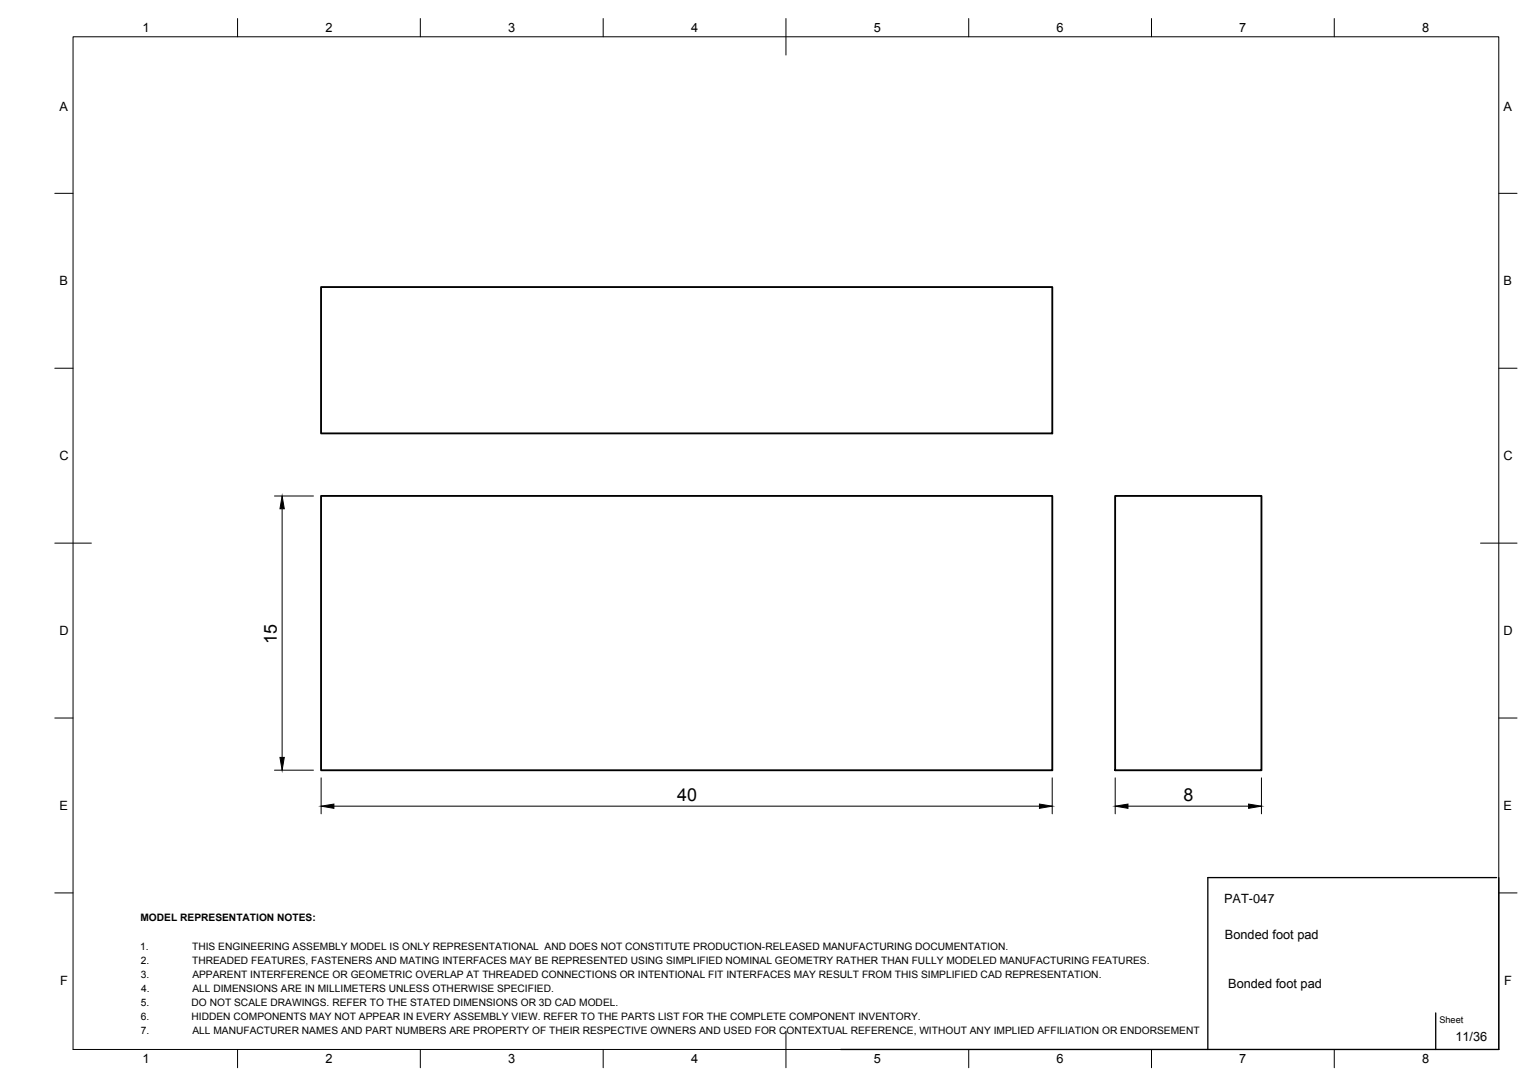
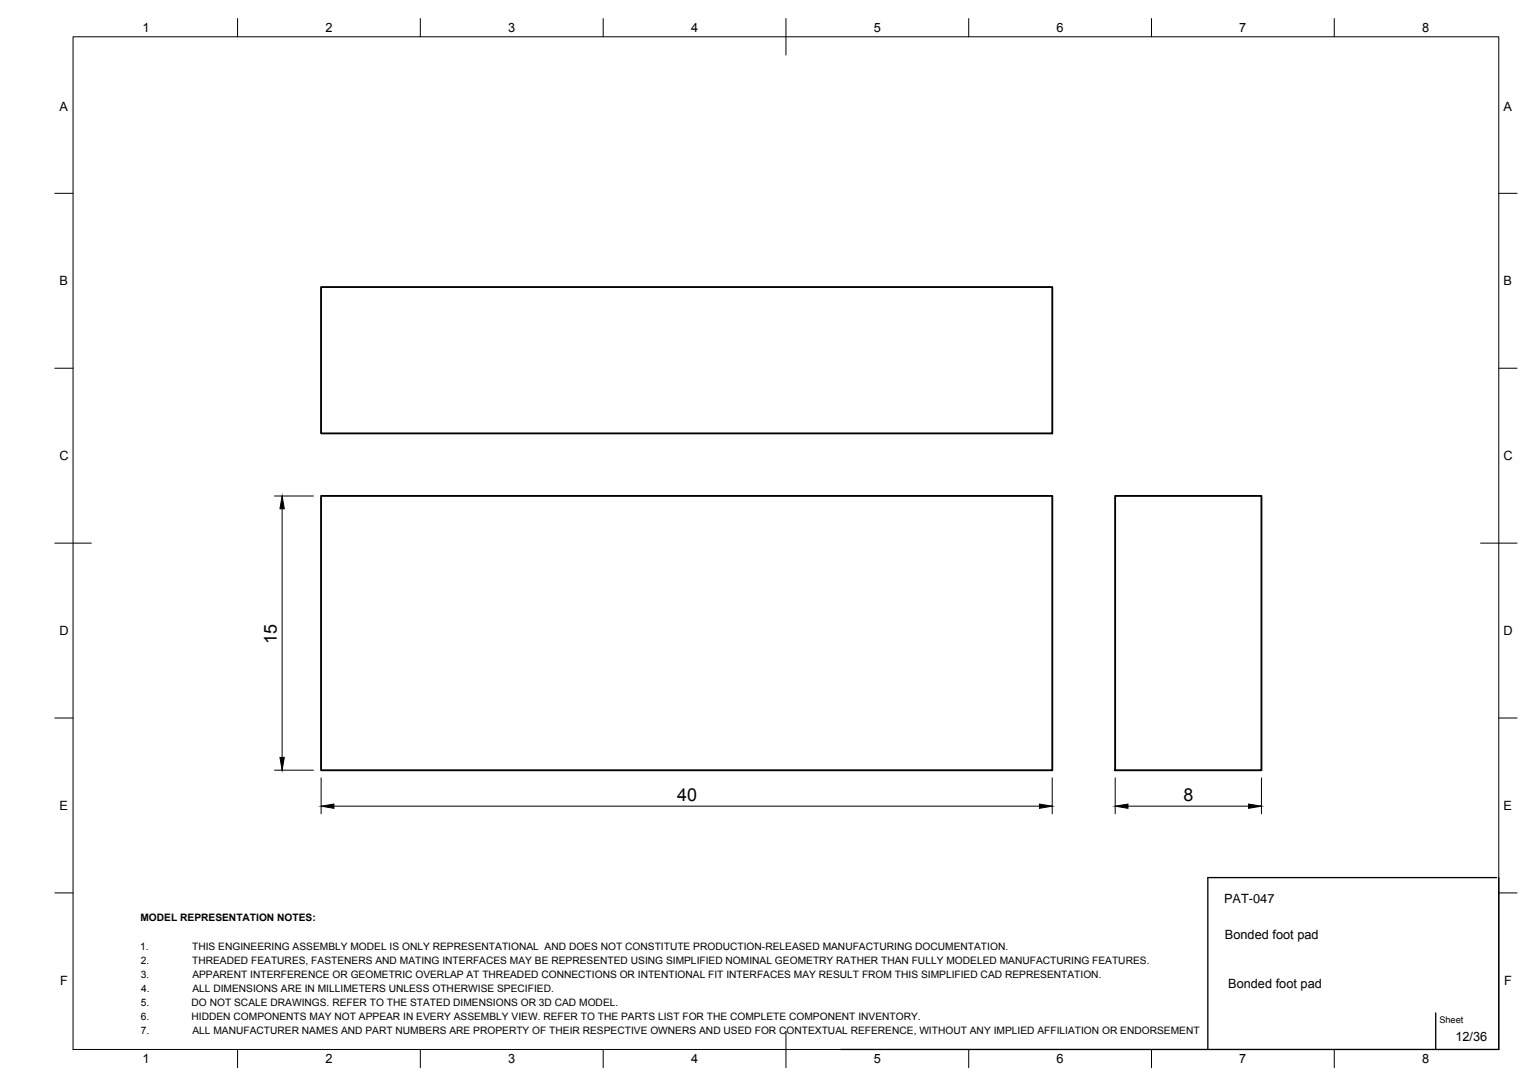
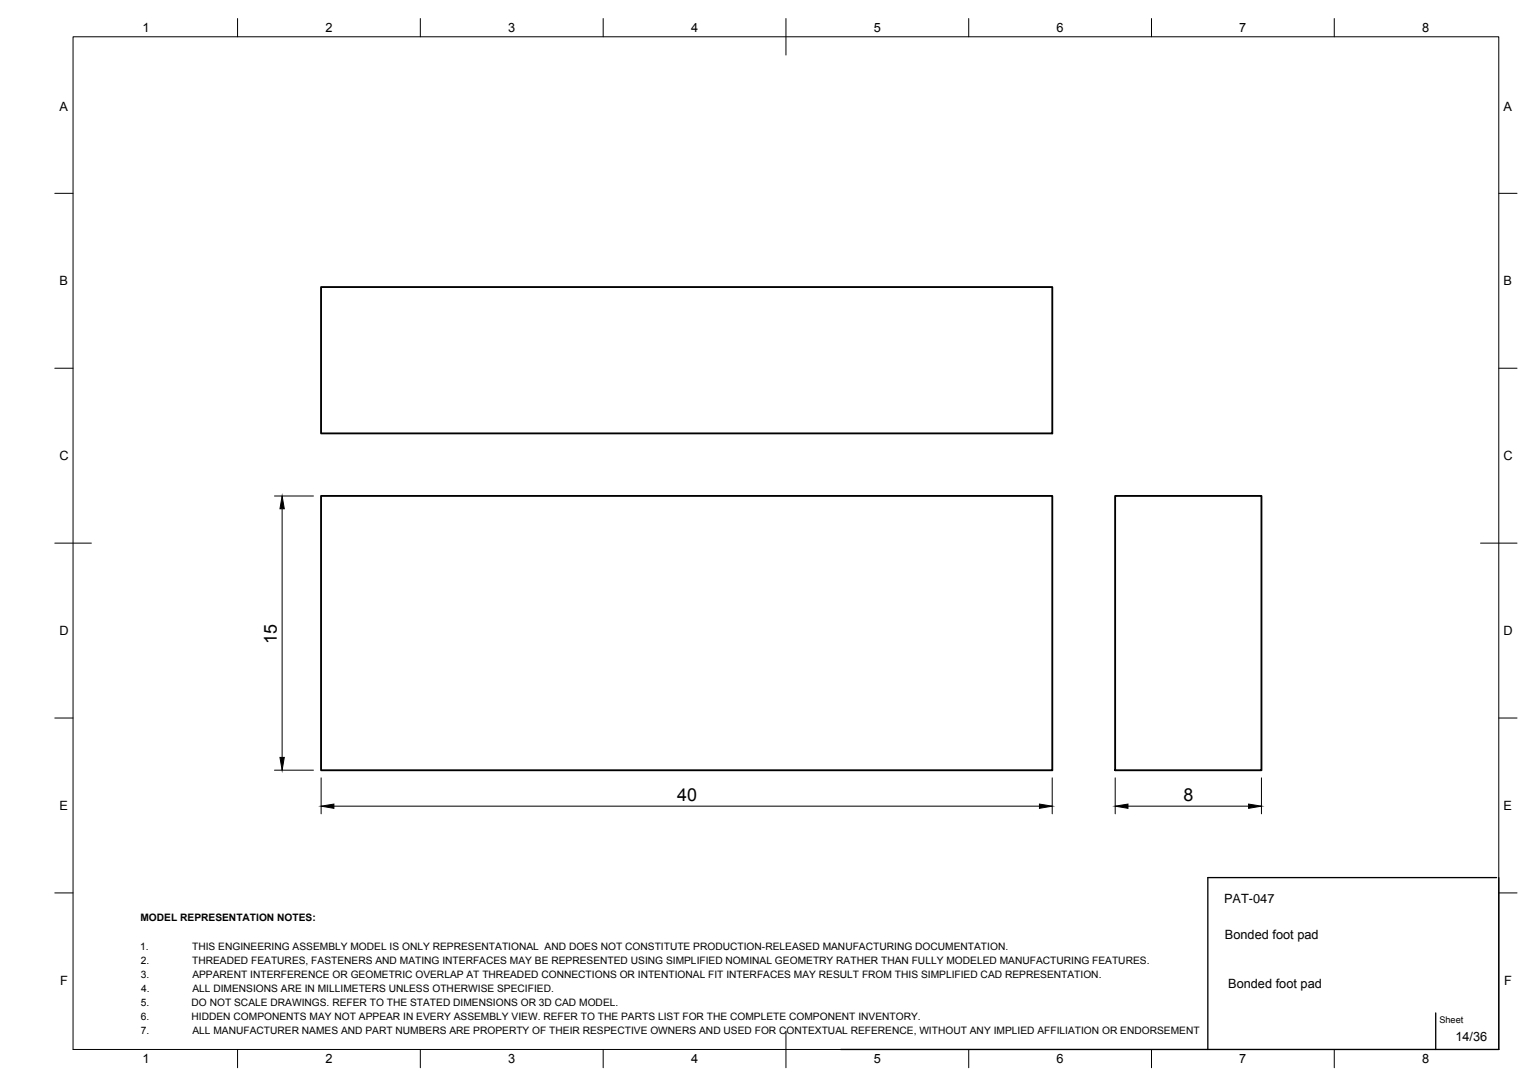
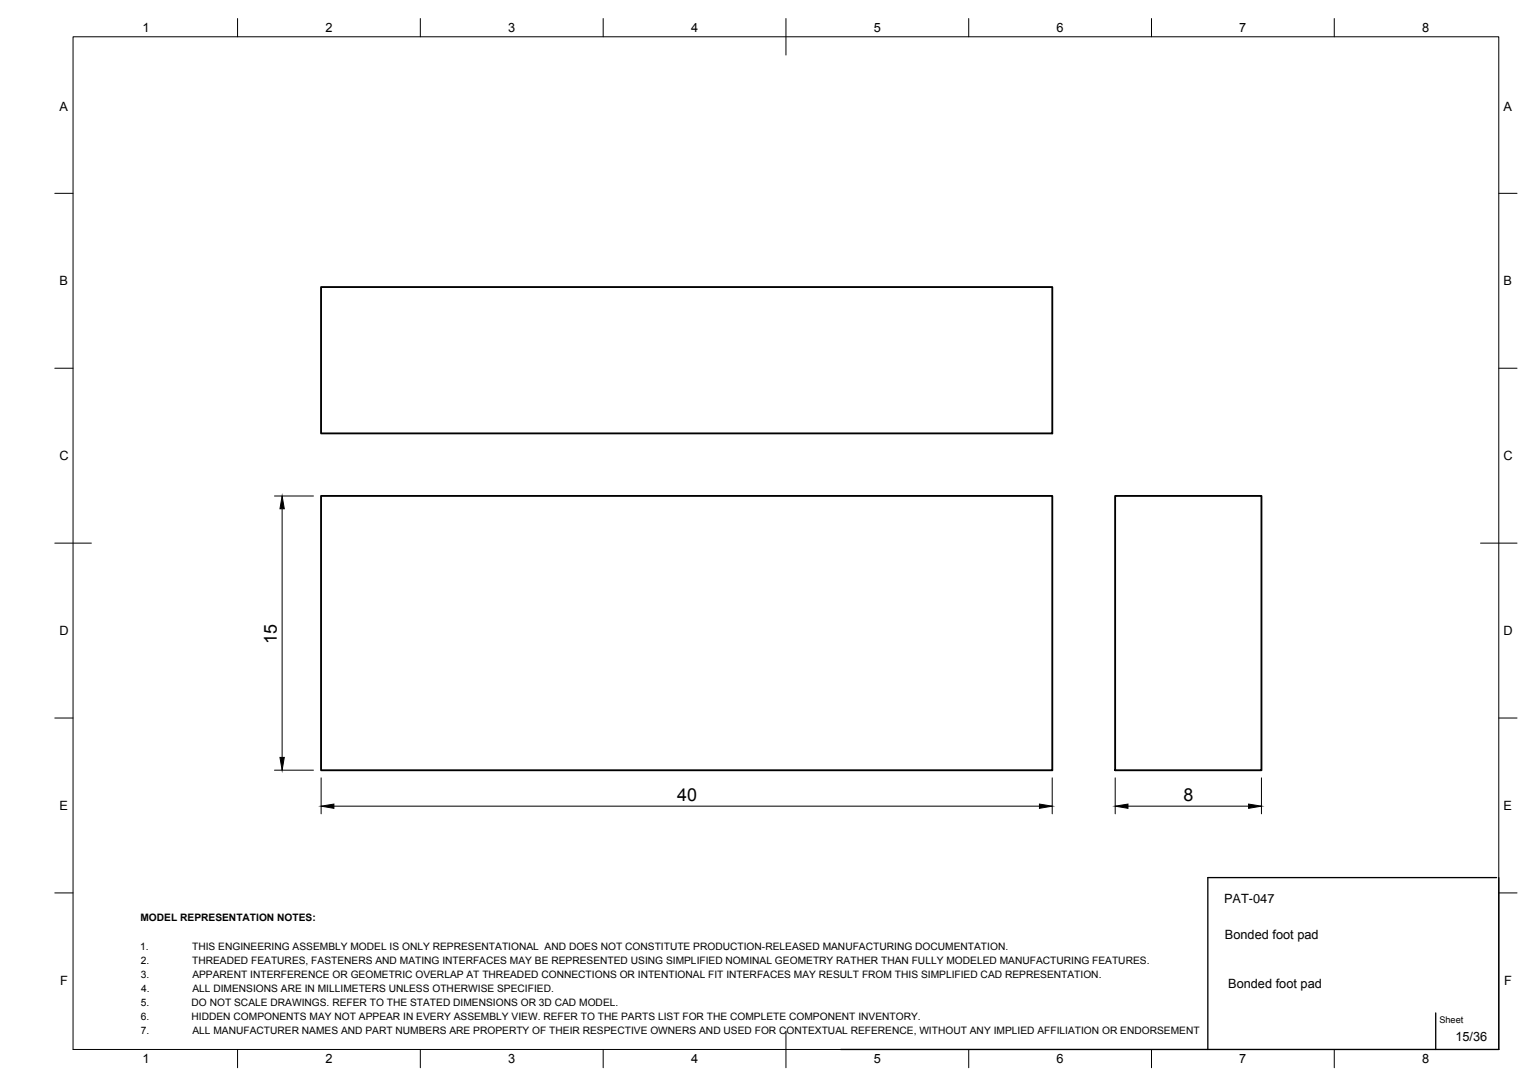
ISO-10303-21;
HEADER;
/* Generated by software containing ST-Developer
 * from STEP Tools, Inc. (www.steptools.com) 
 */

FILE_DESCRIPTION(
/* description */ ('Gravity roller conveyor section'),
/* implementation_level */ '2;1');

FILE_NAME(
/* name */ 'Bonded foot pad.step',
/* time_stamp */ '2026-11-02T07:43:02-08:00',
/* author */ (''),
/* organization */ (''),
/* preprocessor_version */ 'ST-DEVELOPER v20.2',
/* originating_system */ 'Autodesk Translation Framework v15.17.0.0',
/* authorisation */ '');

FILE_SCHEMA (('AUTOMOTIVE_DESIGN { 1 0 10303 214 3 1 1 }'));
ENDSEC;

DATA;
#10=MECHANICAL_DESIGN_GEOMETRIC_PRESENTATION_REPRESENTATION('',(#538),#13821);
#470=SHAPE_REPRESENTATION_RELATIONSHIP('SRR','None',#14007,#504);
#504=ADVANCED_BREP_SHAPE_REPRESENTATION('',(#578),#13794);
#538=STYLED_ITEM('',(#14193),#578);
#578=MANIFOLD_SOLID_BREP('Body1',#7638);
#883=PLANE('',#8325);
#884=PLANE('',#8326);
#885=PLANE('',#8327);
#886=PLANE('',#8328);
#887=PLANE('',#8329);
#888=PLANE('',#8330);
#1220=FACE_OUTER_BOUND('',#1676,.T.);
#1221=FACE_OUTER_BOUND('',#1677,.T.);
#1222=FACE_OUTER_BOUND('',#1678,.T.);
#1223=FACE_OUTER_BOUND('',#1679,.T.);
#1224=FACE_OUTER_BOUND('',#1680,.T.);
#1225=FACE_OUTER_BOUND('',#1681,.T.);
#1676=EDGE_LOOP('',(#6330,#6331,#6332,#6333));
#1677=EDGE_LOOP('',(#6334,#6335,#6336,#6337));
#1678=EDGE_LOOP('',(#6338,#6339,#6340,#6341));
#1679=EDGE_LOOP('',(#6342,#6343,#6344,#6345));
#1680=EDGE_LOOP('',(#6346,#6347,#6348,#6349));
#1681=EDGE_LOOP('',(#6350,#6351,#6352,#6353));
#2440=LINE('',#12409,#3158);
#2441=LINE('',#12411,#3159);
#2442=LINE('',#12413,#3160);
#2443=LINE('',#12414,#3161);
#2444=LINE('',#12417,#3162);
#2445=LINE('',#12419,#3163);
#2446=LINE('',#12420,#3164);
#2447=LINE('',#12423,#3165);
#2448=LINE('',#12425,#3166);
#2449=LINE('',#12426,#3167);
#2450=LINE('',#12428,#3168);
#2451=LINE('',#12429,#3169);
#3158=VECTOR('',#9875,1.);
#3159=VECTOR('',#9876,1.);
#3160=VECTOR('',#9877,1.);
#3161=VECTOR('',#9878,1.);
#3162=VECTOR('',#9881,1.);
#3163=VECTOR('',#9882,1.);
#3164=VECTOR('',#9883,1.);
#3165=VECTOR('',#9886,1.);
#3166=VECTOR('',#9887,1.);
#3167=VECTOR('',#9888,1.);
#3168=VECTOR('',#9891,1.);
#3169=VECTOR('',#9892,1.);
#3964=VERTEX_POINT('',#12407);
#3965=VERTEX_POINT('',#12408);
#3966=VERTEX_POINT('',#12410);
#3967=VERTEX_POINT('',#12412);
#3968=VERTEX_POINT('',#12416);
#3969=VERTEX_POINT('',#12418);
#3970=VERTEX_POINT('',#12422);
#3971=VERTEX_POINT('',#12424);
#4802=EDGE_CURVE('',#3964,#3965,#2440,.T.);
#4803=EDGE_CURVE('',#3965,#3966,#2441,.T.);
#4804=EDGE_CURVE('',#3967,#3966,#2442,.T.);
#4805=EDGE_CURVE('',#3964,#3967,#2443,.T.);
#4806=EDGE_CURVE('',#3968,#3964,#2444,.T.);
#4807=EDGE_CURVE('',#3969,#3967,#2445,.T.);
#4808=EDGE_CURVE('',#3968,#3969,#2446,.T.);
#4809=EDGE_CURVE('',#3970,#3968,#2447,.T.);
#4810=EDGE_CURVE('',#3971,#3969,#2448,.T.);
#4811=EDGE_CURVE('',#3970,#3971,#2449,.T.);
#4812=EDGE_CURVE('',#3965,#3970,#2450,.T.);
#4813=EDGE_CURVE('',#3966,#3971,#2451,.T.);
#6330=ORIENTED_EDGE('',*,*,#4802,.T.);
#6331=ORIENTED_EDGE('',*,*,#4803,.T.);
#6332=ORIENTED_EDGE('',*,*,#4804,.F.);
#6333=ORIENTED_EDGE('',*,*,#4805,.F.);
#6334=ORIENTED_EDGE('',*,*,#4806,.T.);
#6335=ORIENTED_EDGE('',*,*,#4805,.T.);
#6336=ORIENTED_EDGE('',*,*,#4807,.F.);
#6337=ORIENTED_EDGE('',*,*,#4808,.F.);
#6338=ORIENTED_EDGE('',*,*,#4809,.T.);
#6339=ORIENTED_EDGE('',*,*,#4808,.T.);
#6340=ORIENTED_EDGE('',*,*,#4810,.F.);
#6341=ORIENTED_EDGE('',*,*,#4811,.F.);
#6342=ORIENTED_EDGE('',*,*,#4812,.T.);
#6343=ORIENTED_EDGE('',*,*,#4811,.T.);
#6344=ORIENTED_EDGE('',*,*,#4813,.F.);
#6345=ORIENTED_EDGE('',*,*,#4803,.F.);
#6346=ORIENTED_EDGE('',*,*,#4813,.T.);
#6347=ORIENTED_EDGE('',*,*,#4810,.T.);
#6348=ORIENTED_EDGE('',*,*,#4807,.T.);
#6349=ORIENTED_EDGE('',*,*,#4804,.T.);
#6350=ORIENTED_EDGE('',*,*,#4812,.F.);
#6351=ORIENTED_EDGE('',*,*,#4802,.F.);
#6352=ORIENTED_EDGE('',*,*,#4806,.F.);
#6353=ORIENTED_EDGE('',*,*,#4809,.F.);
#7421=ADVANCED_FACE('',(#1220),#883,.T.);
#7422=ADVANCED_FACE('',(#1221),#884,.T.);
#7423=ADVANCED_FACE('',(#1222),#885,.T.);
#7424=ADVANCED_FACE('',(#1223),#886,.T.);
#7425=ADVANCED_FACE('',(#1224),#887,.T.);
#7426=ADVANCED_FACE('',(#1225),#888,.F.);
#7638=CLOSED_SHELL('',(#7421,#7422,#7423,#7424,#7425,#7426));
#8324=AXIS2_PLACEMENT_3D('',#12405,#9871,#9872);
#8325=AXIS2_PLACEMENT_3D('',#12406,#9873,#9874);
#8326=AXIS2_PLACEMENT_3D('',#12415,#9879,#9880);
#8327=AXIS2_PLACEMENT_3D('',#12421,#9884,#9885);
#8328=AXIS2_PLACEMENT_3D('',#12427,#9889,#9890);
#8329=AXIS2_PLACEMENT_3D('',#12430,#9893,#9894);
#8330=AXIS2_PLACEMENT_3D('',#12431,#9895,#9896);
#9871=DIRECTION('axis',(0.,0.,1.));
#9872=DIRECTION('refdir',(1.,0.,0.));
#9873=DIRECTION('center_axis',(0.,1.,0.));
#9874=DIRECTION('ref_axis',(-1.,0.,0.));
#9875=DIRECTION('',(-1.,0.,0.));
#9876=DIRECTION('',(0.,0.,1.));
#9877=DIRECTION('',(-1.,0.,0.));
#9878=DIRECTION('',(0.,0.,1.));
#9879=DIRECTION('center_axis',(1.,0.,0.));
#9880=DIRECTION('ref_axis',(0.,1.,0.));
#9881=DIRECTION('',(0.,1.,0.));
#9882=DIRECTION('',(0.,1.,0.));
#9883=DIRECTION('',(0.,0.,1.));
#9884=DIRECTION('center_axis',(0.,-1.,0.));
#9885=DIRECTION('ref_axis',(1.,0.,0.));
#9886=DIRECTION('',(1.,0.,0.));
#9887=DIRECTION('',(1.,0.,0.));
#9888=DIRECTION('',(0.,0.,1.));
#9889=DIRECTION('center_axis',(-1.,0.,0.));
#9890=DIRECTION('ref_axis',(0.,-1.,0.));
#9891=DIRECTION('',(0.,-1.,0.));
#9892=DIRECTION('',(0.,-1.,0.));
#9893=DIRECTION('center_axis',(0.,0.,1.));
#9894=DIRECTION('ref_axis',(1.,0.,0.));
#9895=DIRECTION('center_axis',(0.,0.,1.));
#9896=DIRECTION('ref_axis',(1.,0.,0.));
#12405=CARTESIAN_POINT('',(0.,0.,0.));
#12406=CARTESIAN_POINT('Origin',(8.,-3.5,-17.6));
#12407=CARTESIAN_POINT('',(8.,-3.5,-17.6));
#12408=CARTESIAN_POINT('',(4.,-3.5,-17.6));
#12409=CARTESIAN_POINT('',(8.,-3.5,-17.6));
#12410=CARTESIAN_POINT('',(4.,-3.5,-16.8));
#12411=CARTESIAN_POINT('',(4.,-3.5,-17.6));
#12412=CARTESIAN_POINT('',(8.,-3.5,-16.8));
#12413=CARTESIAN_POINT('',(8.,-3.5,-16.8));
#12414=CARTESIAN_POINT('',(8.,-3.5,-17.6));
#12415=CARTESIAN_POINT('Origin',(8.,-5.,-17.6));
#12416=CARTESIAN_POINT('',(8.,-5.,-17.6));
#12417=CARTESIAN_POINT('',(8.,-5.,-17.6));
#12418=CARTESIAN_POINT('',(8.,-5.,-16.8));
#12419=CARTESIAN_POINT('',(8.,-5.,-16.8));
#12420=CARTESIAN_POINT('',(8.,-5.,-17.6));
#12421=CARTESIAN_POINT('Origin',(4.,-5.,-17.6));
#12422=CARTESIAN_POINT('',(4.,-5.,-17.6));
#12423=CARTESIAN_POINT('',(4.,-5.,-17.6));
#12424=CARTESIAN_POINT('',(4.,-5.,-16.8));
#12425=CARTESIAN_POINT('',(4.,-5.,-16.8));
#12426=CARTESIAN_POINT('',(4.,-5.,-17.6));
#12427=CARTESIAN_POINT('Origin',(4.,-3.5,-17.6));
#12428=CARTESIAN_POINT('',(4.,-3.5,-17.6));
#12429=CARTESIAN_POINT('',(4.,-3.5,-16.8));
#12430=CARTESIAN_POINT('Origin',(6.,-4.25,-16.8));
#12431=CARTESIAN_POINT('Origin',(6.,-4.25,-17.6));
#13755=UNCERTAINTY_MEASURE_WITH_UNIT(LENGTH_MEASURE(0.001),#13822,
'DISTANCE_ACCURACY_VALUE',
'Maximum model space distance between geometric entities at asserted c
onnectivities');
#13782=UNCERTAINTY_MEASURE_WITH_UNIT(LENGTH_MEASURE(0.001),#13822,
'DISTANCE_ACCURACY_VALUE',
'Maximum model space distance between geometric entities at asserted c
onnectivities');
#13794=(
GEOMETRIC_REPRESENTATION_CONTEXT(3)
GLOBAL_UNCERTAINTY_ASSIGNED_CONTEXT((#13755))
GLOBAL_UNIT_ASSIGNED_CONTEXT((#13822,#13824,#13825))
REPRESENTATION_CONTEXT('','3D')
);
#13821=(
GEOMETRIC_REPRESENTATION_CONTEXT(3)
GLOBAL_UNCERTAINTY_ASSIGNED_CONTEXT((#13782))
GLOBAL_UNIT_ASSIGNED_CONTEXT((#13822,#13824,#13825))
REPRESENTATION_CONTEXT('','3D')
);
#13822=(
LENGTH_UNIT()
NAMED_UNIT(*)
SI_UNIT(.CENTI.,.METRE.)
);
#13824=(
NAMED_UNIT(*)
PLANE_ANGLE_UNIT()
SI_UNIT($,.RADIAN.)
);
#13825=(
NAMED_UNIT(*)
SI_UNIT($,.STERADIAN.)
SOLID_ANGLE_UNIT()
);
#13837=SHAPE_DEFINITION_REPRESENTATION(#13875,#14007);
#13875=PRODUCT_DEFINITION_SHAPE('',$,#14046);
#14007=SHAPE_REPRESENTATION('',(#8324),#13794);
#14034=PRODUCT_DEFINITION_CONTEXT('part definition',#14150,'design');
#14046=PRODUCT_DEFINITION('Bonded foot pad','Bonded foot pad',#14084,#14034);
#14084=PRODUCT_DEFINITION_FORMATION('',$,#14163);
#14150=APPLICATION_CONTEXT(
'Core Data for Automotive Mechanical Design Process');
#14151=PRODUCT_CONTEXT('part definition',#14150,'mechanical');
#14163=PRODUCT('Bonded foot pad','Bonded foot pad','Bonded foot pad',(#14151));
#14193=PRESENTATION_STYLE_ASSIGNMENT((#14198));
#14198=SURFACE_STYLE_USAGE(.BOTH.,#14203);
#14203=SURFACE_SIDE_STYLE('',(#14208));
#14208=SURFACE_STYLE_FILL_AREA(#14213);
#14213=FILL_AREA_STYLE('CAD Library Painted - Graphite',(#14218));
#14218=FILL_AREA_STYLE_COLOUR('CAD Library Painted - Graphite',#14223);
#14223=COLOUR_RGB('CAD Library Painted - Graphite',0.168627450980392,0.192156862745098,
0.231372549019608);
ENDSEC;
END-ISO-10303-21;
